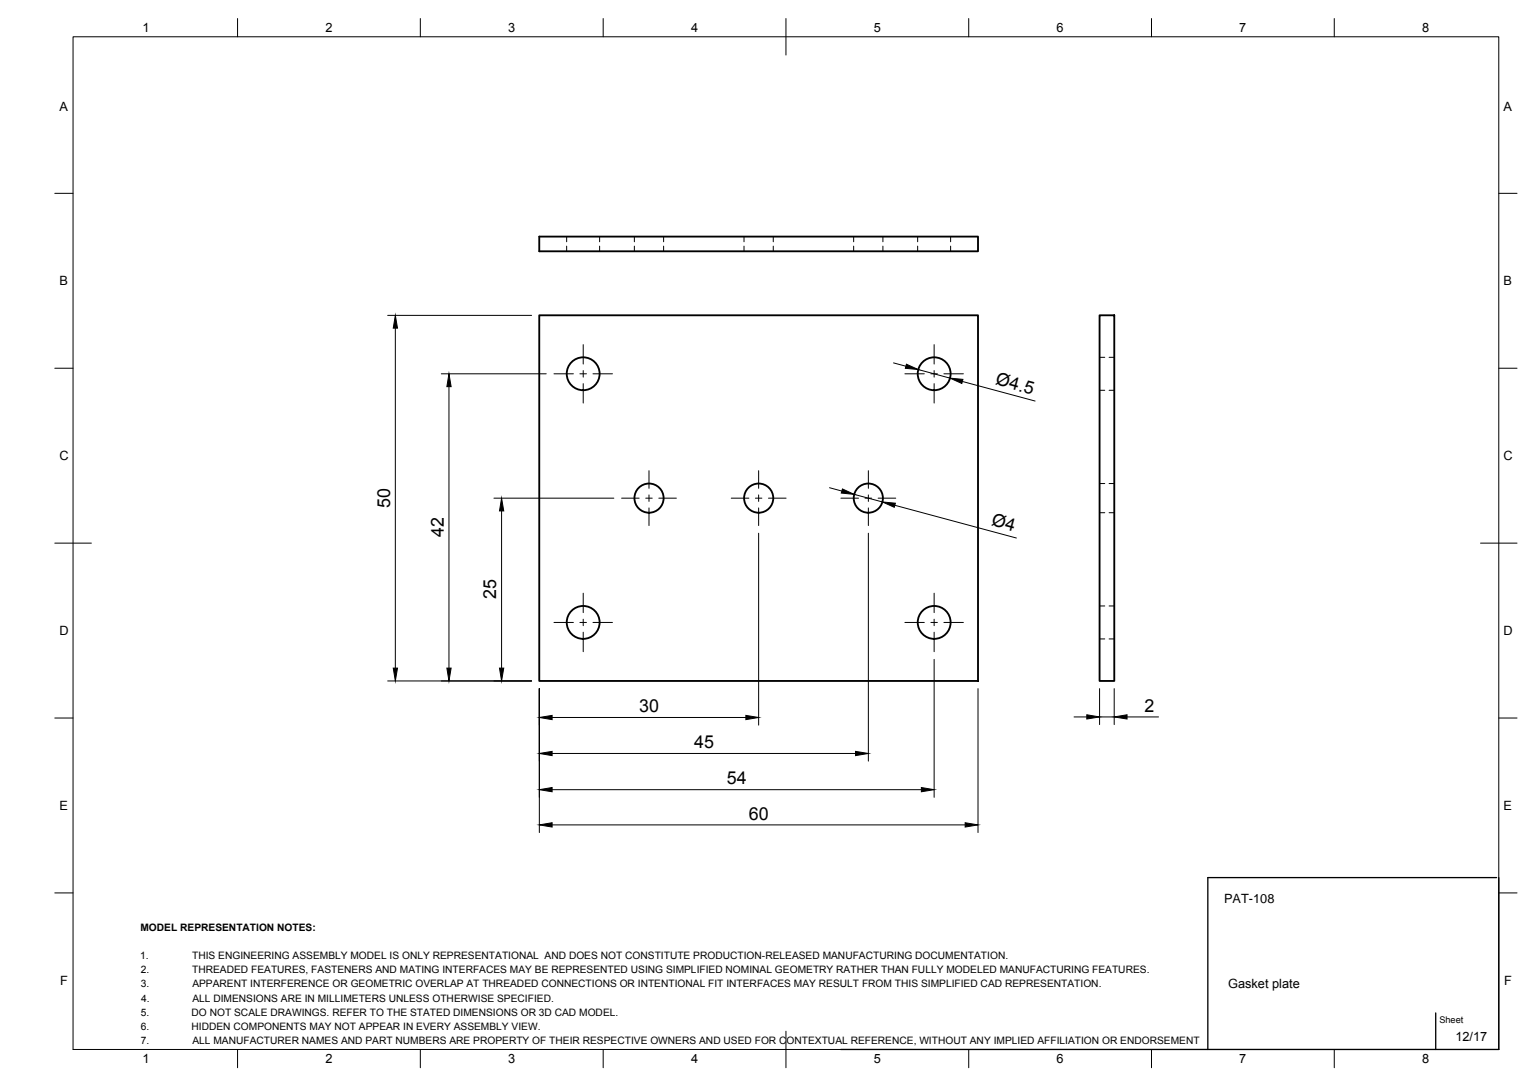
ISO-10303-21;
HEADER;
/* Generated by software containing ST-Developer
 * from STEP Tools, Inc. (www.steptools.com) 
 */

FILE_DESCRIPTION(
/* description */ ('Sub-base valve envelopes and connections'),
/* implementation_level */ '2;1');

FILE_NAME(
/* name */ 'Gasket plate.step',
/* time_stamp */ '2026-10-29T15:55:44-07:00',
/* author */ (''),
/* organization */ (''),
/* preprocessor_version */ 'ST-DEVELOPER v20.2',
/* originating_system */ 'Autodesk Translation Framework v15.17.0.0',
/* authorisation */ '');

FILE_SCHEMA (('AUTOMOTIVE_DESIGN { 1 0 10303 214 3 1 1 }'));
ENDSEC;

DATA;
#10=MECHANICAL_DESIGN_GEOMETRIC_PRESENTATION_REPRESENTATION('',(#126),#6113);
#102=SHAPE_REPRESENTATION_RELATIONSHIP('SRR','None',#6176,#114);
#114=ADVANCED_BREP_SHAPE_REPRESENTATION('',(#138),#6107);
#126=STYLED_ITEM('',(#6329),#138);
#138=MANIFOLD_SOLID_BREP('Body1',#3365);
#231=FACE_BOUND('',#819,.T.);
#232=FACE_BOUND('',#820,.T.);
#233=FACE_BOUND('',#821,.T.);
#234=FACE_BOUND('',#822,.T.);
#235=FACE_BOUND('',#823,.T.);
#236=FACE_BOUND('',#824,.T.);
#237=FACE_BOUND('',#825,.T.);
#238=FACE_BOUND('',#827,.T.);
#239=FACE_BOUND('',#828,.T.);
#240=FACE_BOUND('',#829,.T.);
#241=FACE_BOUND('',#830,.T.);
#242=FACE_BOUND('',#831,.T.);
#243=FACE_BOUND('',#832,.T.);
#244=FACE_BOUND('',#833,.T.);
#344=PLANE('',#3792);
#345=PLANE('',#3793);
#346=PLANE('',#3794);
#347=PLANE('',#3795);
#348=PLANE('',#3796);
#349=PLANE('',#3797);
#519=FACE_OUTER_BOUND('',#807,.T.);
#520=FACE_OUTER_BOUND('',#808,.T.);
#521=FACE_OUTER_BOUND('',#809,.T.);
#522=FACE_OUTER_BOUND('',#810,.T.);
#523=FACE_OUTER_BOUND('',#811,.T.);
#524=FACE_OUTER_BOUND('',#812,.T.);
#525=FACE_OUTER_BOUND('',#813,.T.);
#526=FACE_OUTER_BOUND('',#814,.T.);
#527=FACE_OUTER_BOUND('',#815,.T.);
#528=FACE_OUTER_BOUND('',#816,.T.);
#529=FACE_OUTER_BOUND('',#817,.T.);
#530=FACE_OUTER_BOUND('',#818,.T.);
#531=FACE_OUTER_BOUND('',#826,.T.);
#807=EDGE_LOOP('',(#2807,#2808,#2809,#2810));
#808=EDGE_LOOP('',(#2811,#2812,#2813,#2814));
#809=EDGE_LOOP('',(#2815,#2816,#2817,#2818));
#810=EDGE_LOOP('',(#2819,#2820,#2821,#2822));
#811=EDGE_LOOP('',(#2823,#2824,#2825,#2826));
#812=EDGE_LOOP('',(#2827,#2828,#2829,#2830));
#813=EDGE_LOOP('',(#2831,#2832,#2833,#2834));
#814=EDGE_LOOP('',(#2835,#2836,#2837,#2838));
#815=EDGE_LOOP('',(#2839,#2840,#2841,#2842));
#816=EDGE_LOOP('',(#2843,#2844,#2845,#2846));
#817=EDGE_LOOP('',(#2847,#2848,#2849,#2850));
#818=EDGE_LOOP('',(#2851,#2852,#2853,#2854));
#819=EDGE_LOOP('',(#2855));
#820=EDGE_LOOP('',(#2856));
#821=EDGE_LOOP('',(#2857));
#822=EDGE_LOOP('',(#2858));
#823=EDGE_LOOP('',(#2859));
#824=EDGE_LOOP('',(#2860));
#825=EDGE_LOOP('',(#2861));
#826=EDGE_LOOP('',(#2862,#2863,#2864,#2865));
#827=EDGE_LOOP('',(#2866));
#828=EDGE_LOOP('',(#2867));
#829=EDGE_LOOP('',(#2868));
#830=EDGE_LOOP('',(#2869));
#831=EDGE_LOOP('',(#2870));
#832=EDGE_LOOP('',(#2871));
#833=EDGE_LOOP('',(#2872));
#1045=LINE('',#5774,#1279);
#1046=LINE('',#5780,#1280);
#1047=LINE('',#5786,#1281);
#1048=LINE('',#5792,#1282);
#1049=LINE('',#5798,#1283);
#1050=LINE('',#5804,#1284);
#1051=LINE('',#5810,#1285);
#1052=LINE('',#5815,#1286);
#1053=LINE('',#5817,#1287);
#1054=LINE('',#5819,#1288);
#1055=LINE('',#5820,#1289);
#1056=LINE('',#5823,#1290);
#1057=LINE('',#5825,#1291);
#1058=LINE('',#5826,#1292);
#1059=LINE('',#5829,#1293);
#1060=LINE('',#5831,#1294);
#1061=LINE('',#5832,#1295);
#1062=LINE('',#5834,#1296);
#1063=LINE('',#5835,#1297);
#1279=VECTOR('',#4587,0.225);
#1280=VECTOR('',#4594,0.225);
#1281=VECTOR('',#4601,0.225);
#1282=VECTOR('',#4608,0.225);
#1283=VECTOR('',#4615,0.2);
#1284=VECTOR('',#4622,0.2);
#1285=VECTOR('',#4629,0.2);
#1286=VECTOR('',#4634,1.);
#1287=VECTOR('',#4635,1.);
#1288=VECTOR('',#4636,1.);
#1289=VECTOR('',#4637,1.);
#1290=VECTOR('',#4640,1.);
#1291=VECTOR('',#4641,1.);
#1292=VECTOR('',#4642,1.);
#1293=VECTOR('',#4645,1.);
#1294=VECTOR('',#4646,1.);
#1295=VECTOR('',#4647,1.);
#1296=VECTOR('',#4650,1.);
#1297=VECTOR('',#4651,1.);
#1493=CIRCLE('',#3772,0.225);
#1494=CIRCLE('',#3773,0.225);
#1495=CIRCLE('',#3775,0.225);
#1496=CIRCLE('',#3776,0.225);
#1497=CIRCLE('',#3778,0.225);
#1498=CIRCLE('',#3779,0.225);
#1499=CIRCLE('',#3781,0.225);
#1500=CIRCLE('',#3782,0.225);
#1501=CIRCLE('',#3784,0.2);
#1502=CIRCLE('',#3785,0.2);
#1503=CIRCLE('',#3787,0.2);
#1504=CIRCLE('',#3788,0.2);
#1505=CIRCLE('',#3790,0.2);
#1506=CIRCLE('',#3791,0.2);
#1727=VERTEX_POINT('',#5771);
#1728=VERTEX_POINT('',#5773);
#1729=VERTEX_POINT('',#5777);
#1730=VERTEX_POINT('',#5779);
#1731=VERTEX_POINT('',#5783);
#1732=VERTEX_POINT('',#5785);
#1733=VERTEX_POINT('',#5789);
#1734=VERTEX_POINT('',#5791);
#1735=VERTEX_POINT('',#5795);
#1736=VERTEX_POINT('',#5797);
#1737=VERTEX_POINT('',#5801);
#1738=VERTEX_POINT('',#5803);
#1739=VERTEX_POINT('',#5807);
#1740=VERTEX_POINT('',#5809);
#1741=VERTEX_POINT('',#5813);
#1742=VERTEX_POINT('',#5814);
#1743=VERTEX_POINT('',#5816);
#1744=VERTEX_POINT('',#5818);
#1745=VERTEX_POINT('',#5822);
#1746=VERTEX_POINT('',#5824);
#1747=VERTEX_POINT('',#5828);
#1748=VERTEX_POINT('',#5830);
#2101=EDGE_CURVE('',#1727,#1727,#1493,.T.);
#2102=EDGE_CURVE('',#1727,#1728,#1045,.T.);
#2103=EDGE_CURVE('',#1728,#1728,#1494,.T.);
#2104=EDGE_CURVE('',#1729,#1729,#1495,.T.);
#2105=EDGE_CURVE('',#1729,#1730,#1046,.T.);
#2106=EDGE_CURVE('',#1730,#1730,#1496,.T.);
#2107=EDGE_CURVE('',#1731,#1731,#1497,.T.);
#2108=EDGE_CURVE('',#1731,#1732,#1047,.T.);
#2109=EDGE_CURVE('',#1732,#1732,#1498,.T.);
#2110=EDGE_CURVE('',#1733,#1733,#1499,.T.);
#2111=EDGE_CURVE('',#1733,#1734,#1048,.T.);
#2112=EDGE_CURVE('',#1734,#1734,#1500,.T.);
#2113=EDGE_CURVE('',#1735,#1735,#1501,.T.);
#2114=EDGE_CURVE('',#1735,#1736,#1049,.T.);
#2115=EDGE_CURVE('',#1736,#1736,#1502,.T.);
#2116=EDGE_CURVE('',#1737,#1737,#1503,.T.);
#2117=EDGE_CURVE('',#1737,#1738,#1050,.T.);
#2118=EDGE_CURVE('',#1738,#1738,#1504,.T.);
#2119=EDGE_CURVE('',#1739,#1739,#1505,.T.);
#2120=EDGE_CURVE('',#1739,#1740,#1051,.T.);
#2121=EDGE_CURVE('',#1740,#1740,#1506,.T.);
#2122=EDGE_CURVE('',#1741,#1742,#1052,.T.);
#2123=EDGE_CURVE('',#1742,#1743,#1053,.T.);
#2124=EDGE_CURVE('',#1744,#1743,#1054,.T.);
#2125=EDGE_CURVE('',#1741,#1744,#1055,.T.);
#2126=EDGE_CURVE('',#1745,#1741,#1056,.T.);
#2127=EDGE_CURVE('',#1746,#1744,#1057,.T.);
#2128=EDGE_CURVE('',#1745,#1746,#1058,.T.);
#2129=EDGE_CURVE('',#1747,#1745,#1059,.T.);
#2130=EDGE_CURVE('',#1748,#1746,#1060,.T.);
#2131=EDGE_CURVE('',#1747,#1748,#1061,.T.);
#2132=EDGE_CURVE('',#1742,#1747,#1062,.T.);
#2133=EDGE_CURVE('',#1743,#1748,#1063,.T.);
#2807=ORIENTED_EDGE('',*,*,#2101,.F.);
#2808=ORIENTED_EDGE('',*,*,#2102,.T.);
#2809=ORIENTED_EDGE('',*,*,#2103,.F.);
#2810=ORIENTED_EDGE('',*,*,#2102,.F.);
#2811=ORIENTED_EDGE('',*,*,#2104,.F.);
#2812=ORIENTED_EDGE('',*,*,#2105,.T.);
#2813=ORIENTED_EDGE('',*,*,#2106,.F.);
#2814=ORIENTED_EDGE('',*,*,#2105,.F.);
#2815=ORIENTED_EDGE('',*,*,#2107,.F.);
#2816=ORIENTED_EDGE('',*,*,#2108,.T.);
#2817=ORIENTED_EDGE('',*,*,#2109,.F.);
#2818=ORIENTED_EDGE('',*,*,#2108,.F.);
#2819=ORIENTED_EDGE('',*,*,#2110,.F.);
#2820=ORIENTED_EDGE('',*,*,#2111,.T.);
#2821=ORIENTED_EDGE('',*,*,#2112,.F.);
#2822=ORIENTED_EDGE('',*,*,#2111,.F.);
#2823=ORIENTED_EDGE('',*,*,#2113,.F.);
#2824=ORIENTED_EDGE('',*,*,#2114,.T.);
#2825=ORIENTED_EDGE('',*,*,#2115,.F.);
#2826=ORIENTED_EDGE('',*,*,#2114,.F.);
#2827=ORIENTED_EDGE('',*,*,#2116,.F.);
#2828=ORIENTED_EDGE('',*,*,#2117,.T.);
#2829=ORIENTED_EDGE('',*,*,#2118,.F.);
#2830=ORIENTED_EDGE('',*,*,#2117,.F.);
#2831=ORIENTED_EDGE('',*,*,#2119,.F.);
#2832=ORIENTED_EDGE('',*,*,#2120,.T.);
#2833=ORIENTED_EDGE('',*,*,#2121,.F.);
#2834=ORIENTED_EDGE('',*,*,#2120,.F.);
#2835=ORIENTED_EDGE('',*,*,#2122,.T.);
#2836=ORIENTED_EDGE('',*,*,#2123,.T.);
#2837=ORIENTED_EDGE('',*,*,#2124,.F.);
#2838=ORIENTED_EDGE('',*,*,#2125,.F.);
#2839=ORIENTED_EDGE('',*,*,#2126,.T.);
#2840=ORIENTED_EDGE('',*,*,#2125,.T.);
#2841=ORIENTED_EDGE('',*,*,#2127,.F.);
#2842=ORIENTED_EDGE('',*,*,#2128,.F.);
#2843=ORIENTED_EDGE('',*,*,#2129,.T.);
#2844=ORIENTED_EDGE('',*,*,#2128,.T.);
#2845=ORIENTED_EDGE('',*,*,#2130,.F.);
#2846=ORIENTED_EDGE('',*,*,#2131,.F.);
#2847=ORIENTED_EDGE('',*,*,#2132,.T.);
#2848=ORIENTED_EDGE('',*,*,#2131,.T.);
#2849=ORIENTED_EDGE('',*,*,#2133,.F.);
#2850=ORIENTED_EDGE('',*,*,#2123,.F.);
#2851=ORIENTED_EDGE('',*,*,#2133,.T.);
#2852=ORIENTED_EDGE('',*,*,#2130,.T.);
#2853=ORIENTED_EDGE('',*,*,#2127,.T.);
#2854=ORIENTED_EDGE('',*,*,#2124,.T.);
#2855=ORIENTED_EDGE('',*,*,#2121,.T.);
#2856=ORIENTED_EDGE('',*,*,#2118,.T.);
#2857=ORIENTED_EDGE('',*,*,#2115,.T.);
#2858=ORIENTED_EDGE('',*,*,#2112,.T.);
#2859=ORIENTED_EDGE('',*,*,#2109,.T.);
#2860=ORIENTED_EDGE('',*,*,#2106,.T.);
#2861=ORIENTED_EDGE('',*,*,#2103,.T.);
#2862=ORIENTED_EDGE('',*,*,#2132,.F.);
#2863=ORIENTED_EDGE('',*,*,#2122,.F.);
#2864=ORIENTED_EDGE('',*,*,#2126,.F.);
#2865=ORIENTED_EDGE('',*,*,#2129,.F.);
#2866=ORIENTED_EDGE('',*,*,#2119,.T.);
#2867=ORIENTED_EDGE('',*,*,#2116,.T.);
#2868=ORIENTED_EDGE('',*,*,#2113,.T.);
#2869=ORIENTED_EDGE('',*,*,#2110,.T.);
#2870=ORIENTED_EDGE('',*,*,#2107,.T.);
#2871=ORIENTED_EDGE('',*,*,#2104,.T.);
#2872=ORIENTED_EDGE('',*,*,#2101,.T.);
#3139=CYLINDRICAL_SURFACE('',#3771,0.225);
#3140=CYLINDRICAL_SURFACE('',#3774,0.225);
#3141=CYLINDRICAL_SURFACE('',#3777,0.225);
#3142=CYLINDRICAL_SURFACE('',#3780,0.225);
#3143=CYLINDRICAL_SURFACE('',#3783,0.2);
#3144=CYLINDRICAL_SURFACE('',#3786,0.2);
#3145=CYLINDRICAL_SURFACE('',#3789,0.2);
#3292=ADVANCED_FACE('',(#519),#3139,.F.);
#3293=ADVANCED_FACE('',(#520),#3140,.F.);
#3294=ADVANCED_FACE('',(#521),#3141,.F.);
#3295=ADVANCED_FACE('',(#522),#3142,.F.);
#3296=ADVANCED_FACE('',(#523),#3143,.F.);
#3297=ADVANCED_FACE('',(#524),#3144,.F.);
#3298=ADVANCED_FACE('',(#525),#3145,.F.);
#3299=ADVANCED_FACE('',(#526),#344,.T.);
#3300=ADVANCED_FACE('',(#527),#345,.T.);
#3301=ADVANCED_FACE('',(#528),#346,.T.);
#3302=ADVANCED_FACE('',(#529),#347,.T.);
#3303=ADVANCED_FACE('',(#530,#231,#232,#233,#234,#235,#236,#237),#348,.T.);
#3304=ADVANCED_FACE('',(#531,#238,#239,#240,#241,#242,#243,#244),#349,.F.);
#3365=CLOSED_SHELL('',(#3292,#3293,#3294,#3295,#3296,#3297,#3298,#3299,
#3300,#3301,#3302,#3303,#3304));
#3770=AXIS2_PLACEMENT_3D('',#5769,#4581,#4582);
#3771=AXIS2_PLACEMENT_3D('',#5770,#4583,#4584);
#3772=AXIS2_PLACEMENT_3D('',#5772,#4585,#4586);
#3773=AXIS2_PLACEMENT_3D('',#5775,#4588,#4589);
#3774=AXIS2_PLACEMENT_3D('',#5776,#4590,#4591);
#3775=AXIS2_PLACEMENT_3D('',#5778,#4592,#4593);
#3776=AXIS2_PLACEMENT_3D('',#5781,#4595,#4596);
#3777=AXIS2_PLACEMENT_3D('',#5782,#4597,#4598);
#3778=AXIS2_PLACEMENT_3D('',#5784,#4599,#4600);
#3779=AXIS2_PLACEMENT_3D('',#5787,#4602,#4603);
#3780=AXIS2_PLACEMENT_3D('',#5788,#4604,#4605);
#3781=AXIS2_PLACEMENT_3D('',#5790,#4606,#4607);
#3782=AXIS2_PLACEMENT_3D('',#5793,#4609,#4610);
#3783=AXIS2_PLACEMENT_3D('',#5794,#4611,#4612);
#3784=AXIS2_PLACEMENT_3D('',#5796,#4613,#4614);
#3785=AXIS2_PLACEMENT_3D('',#5799,#4616,#4617);
#3786=AXIS2_PLACEMENT_3D('',#5800,#4618,#4619);
#3787=AXIS2_PLACEMENT_3D('',#5802,#4620,#4621);
#3788=AXIS2_PLACEMENT_3D('',#5805,#4623,#4624);
#3789=AXIS2_PLACEMENT_3D('',#5806,#4625,#4626);
#3790=AXIS2_PLACEMENT_3D('',#5808,#4627,#4628);
#3791=AXIS2_PLACEMENT_3D('',#5811,#4630,#4631);
#3792=AXIS2_PLACEMENT_3D('',#5812,#4632,#4633);
#3793=AXIS2_PLACEMENT_3D('',#5821,#4638,#4639);
#3794=AXIS2_PLACEMENT_3D('',#5827,#4643,#4644);
#3795=AXIS2_PLACEMENT_3D('',#5833,#4648,#4649);
#3796=AXIS2_PLACEMENT_3D('',#5836,#4652,#4653);
#3797=AXIS2_PLACEMENT_3D('',#5837,#4654,#4655);
#4581=DIRECTION('axis',(0.,0.,1.));
#4582=DIRECTION('refdir',(1.,0.,0.));
#4583=DIRECTION('center_axis',(0.,0.,1.));
#4584=DIRECTION('ref_axis',(1.,0.,0.));
#4585=DIRECTION('center_axis',(0.,0.,1.));
#4586=DIRECTION('ref_axis',(1.,0.,0.));
#4587=DIRECTION('',(0.,0.,1.));
#4588=DIRECTION('center_axis',(0.,0.,-1.));
#4589=DIRECTION('ref_axis',(1.,0.,0.));
#4590=DIRECTION('center_axis',(0.,0.,1.));
#4591=DIRECTION('ref_axis',(1.,0.,0.));
#4592=DIRECTION('center_axis',(0.,0.,1.));
#4593=DIRECTION('ref_axis',(1.,0.,0.));
#4594=DIRECTION('',(0.,0.,1.));
#4595=DIRECTION('center_axis',(0.,0.,-1.));
#4596=DIRECTION('ref_axis',(1.,0.,0.));
#4597=DIRECTION('center_axis',(0.,0.,1.));
#4598=DIRECTION('ref_axis',(1.,0.,0.));
#4599=DIRECTION('center_axis',(0.,0.,1.));
#4600=DIRECTION('ref_axis',(1.,0.,0.));
#4601=DIRECTION('',(0.,0.,1.));
#4602=DIRECTION('center_axis',(0.,0.,-1.));
#4603=DIRECTION('ref_axis',(1.,0.,0.));
#4604=DIRECTION('center_axis',(0.,0.,1.));
#4605=DIRECTION('ref_axis',(1.,0.,0.));
#4606=DIRECTION('center_axis',(0.,0.,1.));
#4607=DIRECTION('ref_axis',(1.,0.,0.));
#4608=DIRECTION('',(0.,0.,1.));
#4609=DIRECTION('center_axis',(0.,0.,-1.));
#4610=DIRECTION('ref_axis',(1.,0.,0.));
#4611=DIRECTION('center_axis',(0.,0.,1.));
#4612=DIRECTION('ref_axis',(1.,0.,0.));
#4613=DIRECTION('center_axis',(0.,0.,1.));
#4614=DIRECTION('ref_axis',(1.,0.,0.));
#4615=DIRECTION('',(0.,0.,1.));
#4616=DIRECTION('center_axis',(0.,0.,-1.));
#4617=DIRECTION('ref_axis',(1.,0.,0.));
#4618=DIRECTION('center_axis',(0.,0.,1.));
#4619=DIRECTION('ref_axis',(1.,0.,0.));
#4620=DIRECTION('center_axis',(0.,0.,1.));
#4621=DIRECTION('ref_axis',(1.,0.,0.));
#4622=DIRECTION('',(0.,0.,1.));
#4623=DIRECTION('center_axis',(0.,0.,-1.));
#4624=DIRECTION('ref_axis',(1.,0.,0.));
#4625=DIRECTION('center_axis',(0.,0.,1.));
#4626=DIRECTION('ref_axis',(1.,0.,0.));
#4627=DIRECTION('center_axis',(0.,0.,1.));
#4628=DIRECTION('ref_axis',(1.,0.,0.));
#4629=DIRECTION('',(0.,0.,1.));
#4630=DIRECTION('center_axis',(0.,0.,-1.));
#4631=DIRECTION('ref_axis',(1.,0.,0.));
#4632=DIRECTION('center_axis',(0.,1.,0.));
#4633=DIRECTION('ref_axis',(-1.,0.,0.));
#4634=DIRECTION('',(-1.,0.,0.));
#4635=DIRECTION('',(0.,0.,1.));
#4636=DIRECTION('',(-1.,0.,0.));
#4637=DIRECTION('',(0.,0.,1.));
#4638=DIRECTION('center_axis',(1.,0.,0.));
#4639=DIRECTION('ref_axis',(0.,1.,0.));
#4640=DIRECTION('',(0.,1.,0.));
#4641=DIRECTION('',(0.,1.,0.));
#4642=DIRECTION('',(0.,0.,1.));
#4643=DIRECTION('center_axis',(0.,-1.,0.));
#4644=DIRECTION('ref_axis',(1.,0.,0.));
#4645=DIRECTION('',(1.,0.,0.));
#4646=DIRECTION('',(1.,0.,0.));
#4647=DIRECTION('',(0.,0.,1.));
#4648=DIRECTION('center_axis',(-1.,0.,0.));
#4649=DIRECTION('ref_axis',(0.,-1.,0.));
#4650=DIRECTION('',(0.,-1.,0.));
#4651=DIRECTION('',(0.,-1.,0.));
#4652=DIRECTION('center_axis',(0.,0.,1.));
#4653=DIRECTION('ref_axis',(1.,0.,0.));
#4654=DIRECTION('center_axis',(0.,0.,1.));
#4655=DIRECTION('ref_axis',(1.,0.,0.));
#5769=CARTESIAN_POINT('',(0.,0.,0.));
#5770=CARTESIAN_POINT('Origin',(-2.3,-2.4,1.9));
#5771=CARTESIAN_POINT('',(-2.525,-2.4,2.));
#5772=CARTESIAN_POINT('Origin',(-2.3,-2.4,2.));
#5773=CARTESIAN_POINT('',(-2.525,-2.4,2.2));
#5774=CARTESIAN_POINT('',(-2.525,-2.4,1.9));
#5775=CARTESIAN_POINT('Origin',(-2.3,-2.4,2.2));
#5776=CARTESIAN_POINT('Origin',(-5.7,2.4,1.9));
#5777=CARTESIAN_POINT('',(-5.925,2.4,2.));
#5778=CARTESIAN_POINT('Origin',(-5.7,2.4,2.));
#5779=CARTESIAN_POINT('',(-5.925,2.4,2.2));
#5780=CARTESIAN_POINT('',(-5.925,2.4,1.9));
#5781=CARTESIAN_POINT('Origin',(-5.7,2.4,2.2));
#5782=CARTESIAN_POINT('Origin',(-5.7,-2.4,1.9));
#5783=CARTESIAN_POINT('',(-5.925,-2.4,2.));
#5784=CARTESIAN_POINT('Origin',(-5.7,-2.4,2.));
#5785=CARTESIAN_POINT('',(-5.925,-2.4,2.2));
#5786=CARTESIAN_POINT('',(-5.925,-2.4,1.9));
#5787=CARTESIAN_POINT('Origin',(-5.7,-2.4,2.2));
#5788=CARTESIAN_POINT('Origin',(-2.3,2.4,1.9));
#5789=CARTESIAN_POINT('',(-2.525,2.4,2.));
#5790=CARTESIAN_POINT('Origin',(-2.3,2.4,2.));
#5791=CARTESIAN_POINT('',(-2.525,2.4,2.2));
#5792=CARTESIAN_POINT('',(-2.525,2.4,1.9));
#5793=CARTESIAN_POINT('Origin',(-2.3,2.4,2.2));
#5794=CARTESIAN_POINT('Origin',(-4.,-1.5,1.9));
#5795=CARTESIAN_POINT('',(-4.2,-1.5,2.));
#5796=CARTESIAN_POINT('Origin',(-4.,-1.5,2.));
#5797=CARTESIAN_POINT('',(-4.2,-1.5,2.2));
#5798=CARTESIAN_POINT('',(-4.2,-1.5,1.9));
#5799=CARTESIAN_POINT('Origin',(-4.,-1.5,2.2));
#5800=CARTESIAN_POINT('Origin',(-4.,0.,1.9));
#5801=CARTESIAN_POINT('',(-4.2,-2.44929359829471E-17,2.));
#5802=CARTESIAN_POINT('Origin',(-4.,0.,2.));
#5803=CARTESIAN_POINT('',(-4.2,2.44929359829471E-17,2.2));
#5804=CARTESIAN_POINT('',(-4.2,-2.44929359829471E-17,1.9));
#5805=CARTESIAN_POINT('Origin',(-4.,0.,2.2));
#5806=CARTESIAN_POINT('Origin',(-4.,1.5,1.9));
#5807=CARTESIAN_POINT('',(-4.2,1.5,2.));
#5808=CARTESIAN_POINT('Origin',(-4.,1.5,2.));
#5809=CARTESIAN_POINT('',(-4.2,1.5,2.2));
#5810=CARTESIAN_POINT('',(-4.2,1.5,1.9));
#5811=CARTESIAN_POINT('Origin',(-4.,1.5,2.2));
#5812=CARTESIAN_POINT('Origin',(-1.5,3.,2.));
#5813=CARTESIAN_POINT('',(-1.5,3.,2.));
#5814=CARTESIAN_POINT('',(-6.5,3.,2.));
#5815=CARTESIAN_POINT('',(-1.5,3.,2.));
#5816=CARTESIAN_POINT('',(-6.5,3.,2.2));
#5817=CARTESIAN_POINT('',(-6.5,3.,2.));
#5818=CARTESIAN_POINT('',(-1.5,3.,2.2));
#5819=CARTESIAN_POINT('',(-1.5,3.,2.2));
#5820=CARTESIAN_POINT('',(-1.5,3.,2.));
#5821=CARTESIAN_POINT('Origin',(-1.5,-3.,2.));
#5822=CARTESIAN_POINT('',(-1.5,-3.,2.));
#5823=CARTESIAN_POINT('',(-1.5,-3.,2.));
#5824=CARTESIAN_POINT('',(-1.5,-3.,2.2));
#5825=CARTESIAN_POINT('',(-1.5,-3.,2.2));
#5826=CARTESIAN_POINT('',(-1.5,-3.,2.));
#5827=CARTESIAN_POINT('Origin',(-6.5,-3.,2.));
#5828=CARTESIAN_POINT('',(-6.5,-3.,2.));
#5829=CARTESIAN_POINT('',(-6.5,-3.,2.));
#5830=CARTESIAN_POINT('',(-6.5,-3.,2.2));
#5831=CARTESIAN_POINT('',(-6.5,-3.,2.2));
#5832=CARTESIAN_POINT('',(-6.5,-3.,2.));
#5833=CARTESIAN_POINT('Origin',(-6.5,3.,2.));
#5834=CARTESIAN_POINT('',(-6.5,3.,2.));
#5835=CARTESIAN_POINT('',(-6.5,3.,2.2));
#5836=CARTESIAN_POINT('Origin',(-4.,0.,2.2));
#5837=CARTESIAN_POINT('Origin',(-4.,0.,2.));
#6091=UNCERTAINTY_MEASURE_WITH_UNIT(LENGTH_MEASURE(0.001),#6114,
'DISTANCE_ACCURACY_VALUE',
'Maximum model space distance between geometric entities at asserted c
onnectivities');
#6097=UNCERTAINTY_MEASURE_WITH_UNIT(LENGTH_MEASURE(0.001),#6114,
'DISTANCE_ACCURACY_VALUE',
'Maximum model space distance between geometric entities at asserted c
onnectivities');
#6107=(
GEOMETRIC_REPRESENTATION_CONTEXT(3)
GLOBAL_UNCERTAINTY_ASSIGNED_CONTEXT((#6091))
GLOBAL_UNIT_ASSIGNED_CONTEXT((#6114,#6116,#6117))
REPRESENTATION_CONTEXT('','3D')
);
#6113=(
GEOMETRIC_REPRESENTATION_CONTEXT(3)
GLOBAL_UNCERTAINTY_ASSIGNED_CONTEXT((#6097))
GLOBAL_UNIT_ASSIGNED_CONTEXT((#6114,#6116,#6117))
REPRESENTATION_CONTEXT('','3D')
);
#6114=(
LENGTH_UNIT()
NAMED_UNIT(*)
SI_UNIT(.CENTI.,.METRE.)
);
#6116=(
NAMED_UNIT(*)
PLANE_ANGLE_UNIT()
SI_UNIT($,.RADIAN.)
);
#6117=(
NAMED_UNIT(*)
SI_UNIT($,.STERADIAN.)
SOLID_ANGLE_UNIT()
);
#6127=SHAPE_DEFINITION_REPRESENTATION(#6142,#6176);
#6142=PRODUCT_DEFINITION_SHAPE('',$,#6192);
#6176=SHAPE_REPRESENTATION('',(#3770),#6107);
#6182=PRODUCT_DEFINITION_CONTEXT('part definition',#6229,'design');
#6192=PRODUCT_DEFINITION('Gasket plate','Gasket plate',#6207,
#6182);
#6207=PRODUCT_DEFINITION_FORMATION('',$,#6240);
#6229=APPLICATION_CONTEXT(
'Core Data for Automotive Mechanical Design Process');
#6230=PRODUCT_CONTEXT('part definition',#6229,'mechanical');
#6240=PRODUCT('Gasket plate','Gasket plate','Gasket plate',
(#6230));
#6323=COLOUR_RGB('Off White',0.89,0.88,0.83);
#6324=FILL_AREA_STYLE_COLOUR('',#6323);
#6325=FILL_AREA_STYLE('',(#6324));
#6326=SURFACE_STYLE_FILL_AREA(#6325);
#6327=SURFACE_SIDE_STYLE('',(#6326));
#6328=SURFACE_STYLE_USAGE(.BOTH.,#6327);
#6329=PRESENTATION_STYLE_ASSIGNMENT((#6328));
ENDSEC;
END-ISO-10303-21;
